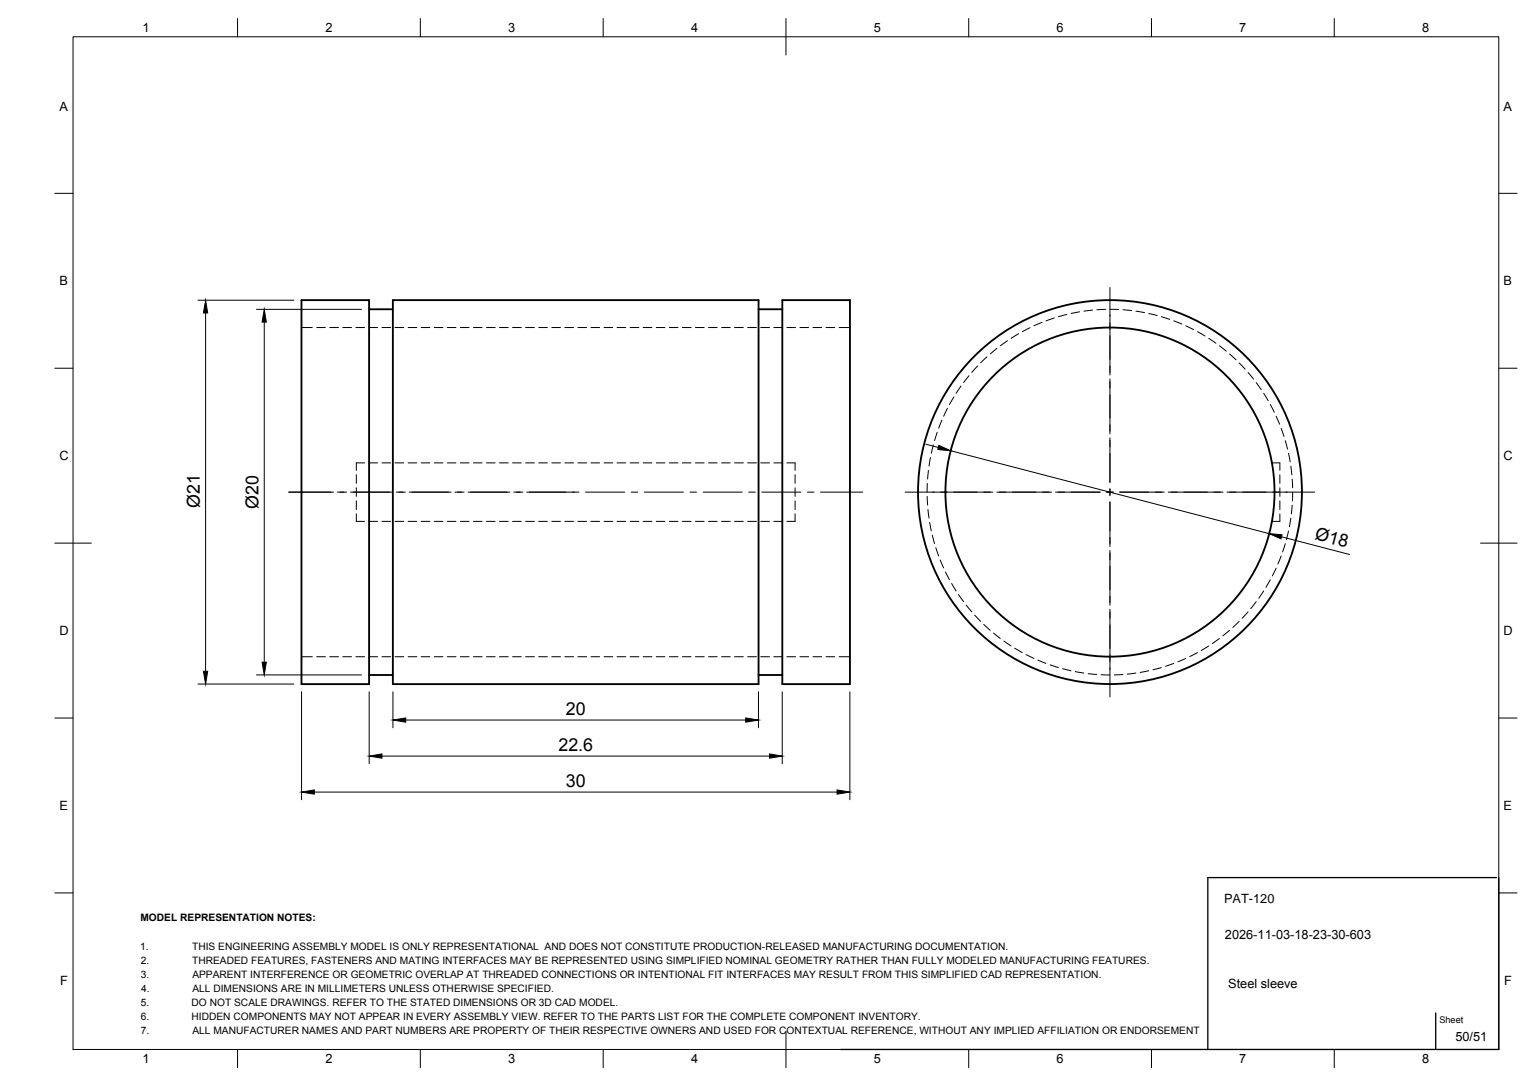
ISO-10303-21;
HEADER;
/* Generated by software containing ST-Developer
 * from STEP Tools, Inc. (www.steptools.com) 
 */

FILE_DESCRIPTION(
/* description */ ('Vibration shaker table dummy'),
/* implementation_level */ '2;1');

FILE_NAME(
/* name */ 'Steel sleeve.step',
/* time_stamp */ '2026-10-27T10:55:14-07:00',
/* author */ (''),
/* organization */ (''),
/* preprocessor_version */ 'ST-DEVELOPER v20.2',
/* originating_system */ 'Autodesk Translation Framework v15.17.0.0',
/* authorisation */ '');

FILE_SCHEMA (('AUTOMOTIVE_DESIGN { 1 0 10303 214 3 1 1 }'));
ENDSEC;

DATA;
#10=MECHANICAL_DESIGN_GEOMETRIC_PRESENTATION_REPRESENTATION('',(#729),#22394);
#637=SHAPE_REPRESENTATION_RELATIONSHIP('SRR','None',#22685,#683);
#683=ADVANCED_BREP_SHAPE_REPRESENTATION('',(#773),#22391);
#729=STYLED_ITEM('',(#22975),#773);
#773=MANIFOLD_SOLID_BREP('Body1',#9249);
#1048=FACE_BOUND('',#2574,.T.);
#1049=FACE_BOUND('',#2577,.T.);
#1050=FACE_BOUND('',#2580,.T.);
#1051=FACE_BOUND('',#2583,.T.);
#1052=FACE_BOUND('',#2586,.T.);
#1053=FACE_BOUND('',#2589,.T.);
#1054=FACE_BOUND('',#2591,.T.);
#1313=PLANE('',#10737);
#1314=PLANE('',#10739);
#1315=PLANE('',#10740);
#1316=PLANE('',#10742);
#1317=PLANE('',#10743);
#1318=PLANE('',#10744);
#1319=PLANE('',#10749);
#1320=PLANE('',#10753);
#1321=PLANE('',#10757);
#1322=PLANE('',#10761);
#1323=PLANE('',#10765);
#1797=FACE_OUTER_BOUND('',#2568,.T.);
#1798=FACE_OUTER_BOUND('',#2569,.T.);
#1799=FACE_OUTER_BOUND('',#2570,.T.);
#1800=FACE_OUTER_BOUND('',#2571,.T.);
#1801=FACE_OUTER_BOUND('',#2572,.T.);
#1802=FACE_OUTER_BOUND('',#2573,.T.);
#1803=FACE_OUTER_BOUND('',#2575,.T.);
#1804=FACE_OUTER_BOUND('',#2576,.T.);
#1805=FACE_OUTER_BOUND('',#2578,.T.);
#1806=FACE_OUTER_BOUND('',#2579,.T.);
#1807=FACE_OUTER_BOUND('',#2581,.T.);
#1808=FACE_OUTER_BOUND('',#2582,.T.);
#1809=FACE_OUTER_BOUND('',#2584,.T.);
#1810=FACE_OUTER_BOUND('',#2585,.T.);
#1811=FACE_OUTER_BOUND('',#2587,.T.);
#1812=FACE_OUTER_BOUND('',#2588,.T.);
#1813=FACE_OUTER_BOUND('',#2590,.T.);
#2568=EDGE_LOOP('',(#8346,#8347,#8348,#8349));
#2569=EDGE_LOOP('',(#8350,#8351,#8352,#8353));
#2570=EDGE_LOOP('',(#8354,#8355,#8356,#8357));
#2571=EDGE_LOOP('',(#8358,#8359,#8360,#8361));
#2572=EDGE_LOOP('',(#8362,#8363,#8364,#8365));
#2573=EDGE_LOOP('',(#8366));
#2574=EDGE_LOOP('',(#8367));
#2575=EDGE_LOOP('',(#8368,#8369,#8370,#8371));
#2576=EDGE_LOOP('',(#8372));
#2577=EDGE_LOOP('',(#8373));
#2578=EDGE_LOOP('',(#8374,#8375,#8376,#8377));
#2579=EDGE_LOOP('',(#8378));
#2580=EDGE_LOOP('',(#8379));
#2581=EDGE_LOOP('',(#8380,#8381,#8382,#8383));
#2582=EDGE_LOOP('',(#8384));
#2583=EDGE_LOOP('',(#8385));
#2584=EDGE_LOOP('',(#8386,#8387,#8388,#8389));
#2585=EDGE_LOOP('',(#8390));
#2586=EDGE_LOOP('',(#8391));
#2587=EDGE_LOOP('',(#8392,#8393,#8394,#8395));
#2588=EDGE_LOOP('',(#8396));
#2589=EDGE_LOOP('',(#8397));
#2590=EDGE_LOOP('',(#8398,#8399,#8400,#8401));
#2591=EDGE_LOOP('',(#8402,#8403,#8404,#8405));
#3191=LINE('',#21983,#3810);
#3192=LINE('',#21985,#3811);
#3193=LINE('',#21986,#3812);
#3194=LINE('',#21989,#3813);
#3195=LINE('',#21991,#3814);
#3196=LINE('',#21992,#3815);
#3197=LINE('',#21997,#3816);
#3198=LINE('',#21998,#3817);
#3199=LINE('',#22000,#3818);
#3200=LINE('',#22001,#3819);
#3201=LINE('',#22011,#3820);
#3202=LINE('',#22018,#3821);
#3203=LINE('',#22025,#3822);
#3204=LINE('',#22032,#3823);
#3205=LINE('',#22039,#3824);
#3206=LINE('',#22044,#3825);
#3810=VECTOR('',#13477,1.);
#3811=VECTOR('',#13478,1.);
#3812=VECTOR('',#13479,1.);
#3813=VECTOR('',#13482,1.);
#3814=VECTOR('',#13483,1.);
#3815=VECTOR('',#13484,1.);
#3816=VECTOR('',#13489,1.);
#3817=VECTOR('',#13490,1.);
#3818=VECTOR('',#13493,1.);
#3819=VECTOR('',#13494,1.);
#3820=VECTOR('',#13507,1.05);
#3821=VECTOR('',#13516,1.);
#3822=VECTOR('',#13525,1.05);
#3823=VECTOR('',#13534,1.);
#3824=VECTOR('',#13543,1.05);
#3825=VECTOR('',#13550,0.9);
#4337=CIRCLE('',#10738,0.9);
#4338=CIRCLE('',#10741,0.9);
#4339=CIRCLE('',#10745,1.05);
#4340=CIRCLE('',#10746,0.9);
#4341=CIRCLE('',#10748,1.05);
#4342=CIRCLE('',#10750,1.);
#4343=CIRCLE('',#10752,1.);
#4344=CIRCLE('',#10754,1.05);
#4345=CIRCLE('',#10756,1.05);
#4346=CIRCLE('',#10758,1.);
#4347=CIRCLE('',#10760,1.);
#4348=CIRCLE('',#10762,1.05);
#4349=CIRCLE('',#10764,1.05);
#4350=CIRCLE('',#10766,0.9);
#5064=VERTEX_POINT('',#21979);
#5065=VERTEX_POINT('',#21980);
#5066=VERTEX_POINT('',#21982);
#5067=VERTEX_POINT('',#21984);
#5068=VERTEX_POINT('',#21988);
#5069=VERTEX_POINT('',#21990);
#5070=VERTEX_POINT('',#21994);
#5071=VERTEX_POINT('',#21996);
#5072=VERTEX_POINT('',#22004);
#5073=VERTEX_POINT('',#22006);
#5074=VERTEX_POINT('',#22009);
#5075=VERTEX_POINT('',#22013);
#5076=VERTEX_POINT('',#22016);
#5077=VERTEX_POINT('',#22020);
#5078=VERTEX_POINT('',#22023);
#5079=VERTEX_POINT('',#22027);
#5080=VERTEX_POINT('',#22030);
#5081=VERTEX_POINT('',#22034);
#5082=VERTEX_POINT('',#22037);
#5083=VERTEX_POINT('',#22041);
#6166=EDGE_CURVE('',#5064,#5065,#4337,.T.);
#6167=EDGE_CURVE('',#5066,#5064,#3191,.T.);
#6168=EDGE_CURVE('',#5067,#5066,#3192,.T.);
#6169=EDGE_CURVE('',#5065,#5067,#3193,.T.);
#6170=EDGE_CURVE('',#5065,#5068,#3194,.T.);
#6171=EDGE_CURVE('',#5069,#5067,#3195,.T.);
#6172=EDGE_CURVE('',#5069,#5068,#3196,.T.);
#6173=EDGE_CURVE('',#5068,#5070,#4338,.T.);
#6174=EDGE_CURVE('',#5071,#5069,#3197,.T.);
#6175=EDGE_CURVE('',#5070,#5071,#3198,.T.);
#6176=EDGE_CURVE('',#5070,#5064,#3199,.T.);
#6177=EDGE_CURVE('',#5071,#5066,#3200,.T.);
#6178=EDGE_CURVE('',#5072,#5072,#4339,.T.);
#6179=EDGE_CURVE('',#5073,#5073,#4340,.T.);
#6180=EDGE_CURVE('',#5074,#5074,#4341,.T.);
#6181=EDGE_CURVE('',#5074,#5072,#3201,.T.);
#6182=EDGE_CURVE('',#5075,#5075,#4342,.T.);
#6183=EDGE_CURVE('',#5076,#5076,#4343,.T.);
#6184=EDGE_CURVE('',#5076,#5075,#3202,.T.);
#6185=EDGE_CURVE('',#5077,#5077,#4344,.T.);
#6186=EDGE_CURVE('',#5078,#5078,#4345,.T.);
#6187=EDGE_CURVE('',#5078,#5077,#3203,.T.);
#6188=EDGE_CURVE('',#5079,#5079,#4346,.T.);
#6189=EDGE_CURVE('',#5080,#5080,#4347,.T.);
#6190=EDGE_CURVE('',#5080,#5079,#3204,.T.);
#6191=EDGE_CURVE('',#5081,#5081,#4348,.T.);
#6192=EDGE_CURVE('',#5082,#5082,#4349,.T.);
#6193=EDGE_CURVE('',#5082,#5081,#3205,.T.);
#6194=EDGE_CURVE('',#5083,#5083,#4350,.T.);
#6195=EDGE_CURVE('',#5083,#5073,#3206,.T.);
#8346=ORIENTED_EDGE('',*,*,#6166,.F.);
#8347=ORIENTED_EDGE('',*,*,#6167,.F.);
#8348=ORIENTED_EDGE('',*,*,#6168,.F.);
#8349=ORIENTED_EDGE('',*,*,#6169,.F.);
#8350=ORIENTED_EDGE('',*,*,#6170,.F.);
#8351=ORIENTED_EDGE('',*,*,#6169,.T.);
#8352=ORIENTED_EDGE('',*,*,#6171,.F.);
#8353=ORIENTED_EDGE('',*,*,#6172,.T.);
#8354=ORIENTED_EDGE('',*,*,#6173,.F.);
#8355=ORIENTED_EDGE('',*,*,#6172,.F.);
#8356=ORIENTED_EDGE('',*,*,#6174,.F.);
#8357=ORIENTED_EDGE('',*,*,#6175,.F.);
#8358=ORIENTED_EDGE('',*,*,#6176,.F.);
#8359=ORIENTED_EDGE('',*,*,#6175,.T.);
#8360=ORIENTED_EDGE('',*,*,#6177,.T.);
#8361=ORIENTED_EDGE('',*,*,#6167,.T.);
#8362=ORIENTED_EDGE('',*,*,#6177,.F.);
#8363=ORIENTED_EDGE('',*,*,#6174,.T.);
#8364=ORIENTED_EDGE('',*,*,#6171,.T.);
#8365=ORIENTED_EDGE('',*,*,#6168,.T.);
#8366=ORIENTED_EDGE('',*,*,#6178,.F.);
#8367=ORIENTED_EDGE('',*,*,#6179,.T.);
#8368=ORIENTED_EDGE('',*,*,#6180,.F.);
#8369=ORIENTED_EDGE('',*,*,#6181,.T.);
#8370=ORIENTED_EDGE('',*,*,#6178,.T.);
#8371=ORIENTED_EDGE('',*,*,#6181,.F.);
#8372=ORIENTED_EDGE('',*,*,#6180,.T.);
#8373=ORIENTED_EDGE('',*,*,#6182,.F.);
#8374=ORIENTED_EDGE('',*,*,#6183,.F.);
#8375=ORIENTED_EDGE('',*,*,#6184,.T.);
#8376=ORIENTED_EDGE('',*,*,#6182,.T.);
#8377=ORIENTED_EDGE('',*,*,#6184,.F.);
#8378=ORIENTED_EDGE('',*,*,#6185,.F.);
#8379=ORIENTED_EDGE('',*,*,#6183,.T.);
#8380=ORIENTED_EDGE('',*,*,#6186,.F.);
#8381=ORIENTED_EDGE('',*,*,#6187,.T.);
#8382=ORIENTED_EDGE('',*,*,#6185,.T.);
#8383=ORIENTED_EDGE('',*,*,#6187,.F.);
#8384=ORIENTED_EDGE('',*,*,#6186,.T.);
#8385=ORIENTED_EDGE('',*,*,#6188,.F.);
#8386=ORIENTED_EDGE('',*,*,#6189,.F.);
#8387=ORIENTED_EDGE('',*,*,#6190,.T.);
#8388=ORIENTED_EDGE('',*,*,#6188,.T.);
#8389=ORIENTED_EDGE('',*,*,#6190,.F.);
#8390=ORIENTED_EDGE('',*,*,#6191,.F.);
#8391=ORIENTED_EDGE('',*,*,#6189,.T.);
#8392=ORIENTED_EDGE('',*,*,#6192,.F.);
#8393=ORIENTED_EDGE('',*,*,#6193,.T.);
#8394=ORIENTED_EDGE('',*,*,#6191,.T.);
#8395=ORIENTED_EDGE('',*,*,#6193,.F.);
#8396=ORIENTED_EDGE('',*,*,#6192,.T.);
#8397=ORIENTED_EDGE('',*,*,#6194,.F.);
#8398=ORIENTED_EDGE('',*,*,#6194,.T.);
#8399=ORIENTED_EDGE('',*,*,#6195,.T.);
#8400=ORIENTED_EDGE('',*,*,#6179,.F.);
#8401=ORIENTED_EDGE('',*,*,#6195,.F.);
#8402=ORIENTED_EDGE('',*,*,#6173,.T.);
#8403=ORIENTED_EDGE('',*,*,#6176,.T.);
#8404=ORIENTED_EDGE('',*,*,#6166,.T.);
#8405=ORIENTED_EDGE('',*,*,#6170,.T.);
#8696=CYLINDRICAL_SURFACE('',#10747,1.05);
#8697=CYLINDRICAL_SURFACE('',#10751,1.);
#8698=CYLINDRICAL_SURFACE('',#10755,1.05);
#8699=CYLINDRICAL_SURFACE('',#10759,1.);
#8700=CYLINDRICAL_SURFACE('',#10763,1.05);
#8701=CYLINDRICAL_SURFACE('',#10767,0.9);
#9162=ADVANCED_FACE('',(#1797),#1313,.F.);
#9163=ADVANCED_FACE('',(#1798),#1314,.F.);
#9164=ADVANCED_FACE('',(#1799),#1315,.F.);
#9165=ADVANCED_FACE('',(#1800),#1316,.F.);
#9166=ADVANCED_FACE('',(#1801),#1317,.F.);
#9167=ADVANCED_FACE('',(#1802,#1048),#1318,.T.);
#9168=ADVANCED_FACE('',(#1803),#8696,.T.);
#9169=ADVANCED_FACE('',(#1804,#1049),#1319,.T.);
#9170=ADVANCED_FACE('',(#1805),#8697,.T.);
#9171=ADVANCED_FACE('',(#1806,#1050),#1320,.T.);
#9172=ADVANCED_FACE('',(#1807),#8698,.T.);
#9173=ADVANCED_FACE('',(#1808,#1051),#1321,.T.);
#9174=ADVANCED_FACE('',(#1809),#8699,.T.);
#9175=ADVANCED_FACE('',(#1810,#1052),#1322,.T.);
#9176=ADVANCED_FACE('',(#1811),#8700,.T.);
#9177=ADVANCED_FACE('',(#1812,#1053),#1323,.T.);
#9178=ADVANCED_FACE('',(#1813,#1054),#8701,.F.);
#9249=CLOSED_SHELL('',(#9162,#9163,#9164,#9165,#9166,#9167,#9168,#9169,
#9170,#9171,#9172,#9173,#9174,#9175,#9176,#9177,#9178));
#10736=AXIS2_PLACEMENT_3D('',#21977,#13471,#13472);
#10737=AXIS2_PLACEMENT_3D('',#21978,#13473,#13474);
#10738=AXIS2_PLACEMENT_3D('',#21981,#13475,#13476);
#10739=AXIS2_PLACEMENT_3D('',#21987,#13480,#13481);
#10740=AXIS2_PLACEMENT_3D('',#21993,#13485,#13486);
#10741=AXIS2_PLACEMENT_3D('',#21995,#13487,#13488);
#10742=AXIS2_PLACEMENT_3D('',#21999,#13491,#13492);
#10743=AXIS2_PLACEMENT_3D('',#22002,#13495,#13496);
#10744=AXIS2_PLACEMENT_3D('',#22003,#13497,#13498);
#10745=AXIS2_PLACEMENT_3D('',#22005,#13499,#13500);
#10746=AXIS2_PLACEMENT_3D('',#22007,#13501,#13502);
#10747=AXIS2_PLACEMENT_3D('',#22008,#13503,#13504);
#10748=AXIS2_PLACEMENT_3D('',#22010,#13505,#13506);
#10749=AXIS2_PLACEMENT_3D('',#22012,#13508,#13509);
#10750=AXIS2_PLACEMENT_3D('',#22014,#13510,#13511);
#10751=AXIS2_PLACEMENT_3D('',#22015,#13512,#13513);
#10752=AXIS2_PLACEMENT_3D('',#22017,#13514,#13515);
#10753=AXIS2_PLACEMENT_3D('',#22019,#13517,#13518);
#10754=AXIS2_PLACEMENT_3D('',#22021,#13519,#13520);
#10755=AXIS2_PLACEMENT_3D('',#22022,#13521,#13522);
#10756=AXIS2_PLACEMENT_3D('',#22024,#13523,#13524);
#10757=AXIS2_PLACEMENT_3D('',#22026,#13526,#13527);
#10758=AXIS2_PLACEMENT_3D('',#22028,#13528,#13529);
#10759=AXIS2_PLACEMENT_3D('',#22029,#13530,#13531);
#10760=AXIS2_PLACEMENT_3D('',#22031,#13532,#13533);
#10761=AXIS2_PLACEMENT_3D('',#22033,#13535,#13536);
#10762=AXIS2_PLACEMENT_3D('',#22035,#13537,#13538);
#10763=AXIS2_PLACEMENT_3D('',#22036,#13539,#13540);
#10764=AXIS2_PLACEMENT_3D('',#22038,#13541,#13542);
#10765=AXIS2_PLACEMENT_3D('',#22040,#13544,#13545);
#10766=AXIS2_PLACEMENT_3D('',#22042,#13546,#13547);
#10767=AXIS2_PLACEMENT_3D('',#22043,#13548,#13549);
#13471=DIRECTION('axis',(0.,0.,1.));
#13472=DIRECTION('refdir',(1.,0.,0.));
#13473=DIRECTION('center_axis',(0.,1.,0.));
#13474=DIRECTION('ref_axis',(0.,0.,1.));
#13475=DIRECTION('center_axis',(0.,-1.,0.));
#13476=DIRECTION('ref_axis',(1.,0.,0.));
#13477=DIRECTION('',(-1.,0.,0.));
#13478=DIRECTION('',(0.,0.,-1.));
#13479=DIRECTION('',(1.,0.,0.));
#13480=DIRECTION('center_axis',(0.,0.,1.));
#13481=DIRECTION('ref_axis',(1.,0.,0.));
#13482=DIRECTION('',(0.,-1.,0.));
#13483=DIRECTION('',(0.,1.,0.));
#13484=DIRECTION('',(-1.,0.,0.));
#13485=DIRECTION('center_axis',(0.,-1.,0.));
#13486=DIRECTION('ref_axis',(0.,0.,-1.));
#13487=DIRECTION('center_axis',(0.,1.,0.));
#13488=DIRECTION('ref_axis',(1.,0.,0.));
#13489=DIRECTION('',(0.,0.,1.));
#13490=DIRECTION('',(1.,0.,0.));
#13491=DIRECTION('center_axis',(0.,0.,-1.));
#13492=DIRECTION('ref_axis',(-1.,0.,0.));
#13493=DIRECTION('',(0.,1.,0.));
#13494=DIRECTION('',(0.,1.,0.));
#13495=DIRECTION('center_axis',(1.,0.,0.));
#13496=DIRECTION('ref_axis',(0.,0.,-1.));
#13497=DIRECTION('center_axis',(0.,1.,0.));
#13498=DIRECTION('ref_axis',(0.,0.,1.));
#13499=DIRECTION('center_axis',(0.,-1.,0.));
#13500=DIRECTION('ref_axis',(1.,0.,0.));
#13501=DIRECTION('center_axis',(0.,-1.,0.));
#13502=DIRECTION('ref_axis',(1.,0.,0.));
#13503=DIRECTION('center_axis',(0.,-1.,0.));
#13504=DIRECTION('ref_axis',(1.,0.,0.));
#13505=DIRECTION('center_axis',(0.,-1.,0.));
#13506=DIRECTION('ref_axis',(1.,0.,0.));
#13507=DIRECTION('',(0.,1.,0.));
#13508=DIRECTION('center_axis',(0.,-1.,0.));
#13509=DIRECTION('ref_axis',(0.,0.,-1.));
#13510=DIRECTION('center_axis',(0.,-1.,0.));
#13511=DIRECTION('ref_axis',(1.,0.,0.));
#13512=DIRECTION('center_axis',(0.,-1.,0.));
#13513=DIRECTION('ref_axis',(1.,0.,0.));
#13514=DIRECTION('center_axis',(0.,-1.,0.));
#13515=DIRECTION('ref_axis',(1.,0.,0.));
#13516=DIRECTION('',(0.,1.,0.));
#13517=DIRECTION('center_axis',(0.,1.,0.));
#13518=DIRECTION('ref_axis',(0.,0.,1.));
#13519=DIRECTION('center_axis',(0.,-1.,0.));
#13520=DIRECTION('ref_axis',(1.,0.,0.));
#13521=DIRECTION('center_axis',(0.,-1.,0.));
#13522=DIRECTION('ref_axis',(1.,0.,0.));
#13523=DIRECTION('center_axis',(0.,-1.,0.));
#13524=DIRECTION('ref_axis',(1.,0.,0.));
#13525=DIRECTION('',(0.,1.,0.));
#13526=DIRECTION('center_axis',(0.,-1.,0.));
#13527=DIRECTION('ref_axis',(0.,0.,-1.));
#13528=DIRECTION('center_axis',(0.,-1.,0.));
#13529=DIRECTION('ref_axis',(1.,0.,0.));
#13530=DIRECTION('center_axis',(0.,-1.,0.));
#13531=DIRECTION('ref_axis',(1.,0.,0.));
#13532=DIRECTION('center_axis',(0.,-1.,0.));
#13533=DIRECTION('ref_axis',(1.,0.,0.));
#13534=DIRECTION('',(0.,1.,0.));
#13535=DIRECTION('center_axis',(0.,1.,0.));
#13536=DIRECTION('ref_axis',(0.,0.,1.));
#13537=DIRECTION('center_axis',(0.,-1.,0.));
#13538=DIRECTION('ref_axis',(1.,0.,0.));
#13539=DIRECTION('center_axis',(0.,-1.,0.));
#13540=DIRECTION('ref_axis',(1.,0.,0.));
#13541=DIRECTION('center_axis',(0.,-1.,0.));
#13542=DIRECTION('ref_axis',(1.,0.,0.));
#13543=DIRECTION('',(0.,1.,0.));
#13544=DIRECTION('center_axis',(0.,-1.,0.));
#13545=DIRECTION('ref_axis',(0.,0.,-1.));
#13546=DIRECTION('center_axis',(0.,-1.,0.));
#13547=DIRECTION('ref_axis',(1.,0.,0.));
#13548=DIRECTION('center_axis',(0.,-1.,0.));
#13549=DIRECTION('ref_axis',(1.,0.,0.));
#13550=DIRECTION('',(0.,1.,0.));
#21977=CARTESIAN_POINT('',(0.,0.,0.));
#21978=CARTESIAN_POINT('Origin',(0.75,1.2,0.));
#21979=CARTESIAN_POINT('',(0.885663593019381,1.2,-0.16));
#21980=CARTESIAN_POINT('',(0.885663593019381,1.2,0.16));
#21981=CARTESIAN_POINT('Origin',(0.,1.2,0.));
#21982=CARTESIAN_POINT('',(0.93,1.2,-0.16));
#21983=CARTESIAN_POINT('',(0.93,1.2,-0.16));
#21984=CARTESIAN_POINT('',(0.93,1.2,0.16));
#21985=CARTESIAN_POINT('',(0.93,1.2,0.16));
#21986=CARTESIAN_POINT('',(0.57,1.2,0.16));
#21987=CARTESIAN_POINT('Origin',(0.57,0.,0.16));
#21988=CARTESIAN_POINT('',(0.885663593019381,-1.2,0.16));
#21989=CARTESIAN_POINT('',(0.885663593019381,0.,0.16));
#21990=CARTESIAN_POINT('',(0.93,-1.2,0.16));
#21991=CARTESIAN_POINT('',(0.93,0.,0.16));
#21992=CARTESIAN_POINT('',(0.57,-1.2,0.16));
#21993=CARTESIAN_POINT('Origin',(0.75,-1.2,0.));
#21994=CARTESIAN_POINT('',(0.885663593019381,-1.2,-0.16));
#21995=CARTESIAN_POINT('Origin',(0.,-1.2,0.));
#21996=CARTESIAN_POINT('',(0.93,-1.2,-0.16));
#21997=CARTESIAN_POINT('',(0.93,-1.2,0.16));
#21998=CARTESIAN_POINT('',(0.93,-1.2,-0.16));
#21999=CARTESIAN_POINT('Origin',(0.93,0.,-0.16));
#22000=CARTESIAN_POINT('',(0.885663593019381,0.,-0.16));
#22001=CARTESIAN_POINT('',(0.93,0.,-0.16));
#22002=CARTESIAN_POINT('Origin',(0.93,0.,0.16));
#22003=CARTESIAN_POINT('Origin',(1.05,1.5,0.));
#22004=CARTESIAN_POINT('',(-1.05,1.5,-1.28587913910472E-16));
#22005=CARTESIAN_POINT('Origin',(0.,1.5,0.));
#22006=CARTESIAN_POINT('',(-0.9,1.5,-1.10218211923262E-16));
#22007=CARTESIAN_POINT('Origin',(0.,1.5,0.));
#22008=CARTESIAN_POINT('Origin',(0.,1.315,0.));
#22009=CARTESIAN_POINT('',(-1.05,1.13,-1.28587913910472E-16));
#22010=CARTESIAN_POINT('Origin',(0.,1.13,0.));
#22011=CARTESIAN_POINT('',(-1.05,1.315,-1.28587913910472E-16));
#22012=CARTESIAN_POINT('Origin',(1.,1.13,0.));
#22013=CARTESIAN_POINT('',(-1.,1.13,-1.22464679914735E-16));
#22014=CARTESIAN_POINT('Origin',(0.,1.13,0.));
#22015=CARTESIAN_POINT('Origin',(0.,1.065,0.));
#22016=CARTESIAN_POINT('',(-1.,1.,-1.22464679914735E-16));
#22017=CARTESIAN_POINT('Origin',(0.,1.,0.));
#22018=CARTESIAN_POINT('',(-1.,1.065,-1.22464679914735E-16));
#22019=CARTESIAN_POINT('Origin',(1.05,1.,0.));
#22020=CARTESIAN_POINT('',(-1.05,1.,-1.28587913910472E-16));
#22021=CARTESIAN_POINT('Origin',(0.,1.,0.));
#22022=CARTESIAN_POINT('Origin',(0.,0.,0.));
#22023=CARTESIAN_POINT('',(-1.05,-1.,-1.28587913910472E-16));
#22024=CARTESIAN_POINT('Origin',(0.,-1.,0.));
#22025=CARTESIAN_POINT('',(-1.05,0.,-1.28587913910472E-16));
#22026=CARTESIAN_POINT('Origin',(1.,-1.,0.));
#22027=CARTESIAN_POINT('',(-1.,-1.,-1.22464679914735E-16));
#22028=CARTESIAN_POINT('Origin',(0.,-1.,0.));
#22029=CARTESIAN_POINT('Origin',(0.,-1.065,0.));
#22030=CARTESIAN_POINT('',(-1.,-1.13,-1.22464679914735E-16));
#22031=CARTESIAN_POINT('Origin',(0.,-1.13,0.));
#22032=CARTESIAN_POINT('',(-1.,-1.065,-1.22464679914735E-16));
#22033=CARTESIAN_POINT('Origin',(1.05,-1.13,0.));
#22034=CARTESIAN_POINT('',(-1.05,-1.13,-1.28587913910472E-16));
#22035=CARTESIAN_POINT('Origin',(0.,-1.13,0.));
#22036=CARTESIAN_POINT('Origin',(0.,-1.315,0.));
#22037=CARTESIAN_POINT('',(-1.05,-1.5,-1.28587913910472E-16));
#22038=CARTESIAN_POINT('Origin',(0.,-1.5,0.));
#22039=CARTESIAN_POINT('',(-1.05,-1.315,-1.28587913910472E-16));
#22040=CARTESIAN_POINT('Origin',(0.9,-1.5,0.));
#22041=CARTESIAN_POINT('',(-0.9,-1.5,-1.10218211923262E-16));
#22042=CARTESIAN_POINT('Origin',(0.,-1.5,0.));
#22043=CARTESIAN_POINT('Origin',(0.,0.,0.));
#22044=CARTESIAN_POINT('',(-0.9,0.,-1.10218211923262E-16));
#22340=UNCERTAINTY_MEASURE_WITH_UNIT(LENGTH_MEASURE(0.001),#22395,
'DISTANCE_ACCURACY_VALUE',
'Maximum model space distance between geometric entities at asserted c
onnectivities');
#22343=UNCERTAINTY_MEASURE_WITH_UNIT(LENGTH_MEASURE(0.001),#22395,
'DISTANCE_ACCURACY_VALUE',
'Maximum model space distance between geometric entities at asserted c
onnectivities');
#22391=(
GEOMETRIC_REPRESENTATION_CONTEXT(3)
GLOBAL_UNCERTAINTY_ASSIGNED_CONTEXT((#22340))
GLOBAL_UNIT_ASSIGNED_CONTEXT((#22395,#22397,#22398))
REPRESENTATION_CONTEXT('','3D')
);
#22394=(
GEOMETRIC_REPRESENTATION_CONTEXT(3)
GLOBAL_UNCERTAINTY_ASSIGNED_CONTEXT((#22343))
GLOBAL_UNIT_ASSIGNED_CONTEXT((#22395,#22397,#22398))
REPRESENTATION_CONTEXT('','3D')
);
#22395=(
LENGTH_UNIT()
NAMED_UNIT(*)
SI_UNIT(.CENTI.,.METRE.)
);
#22397=(
NAMED_UNIT(*)
PLANE_ANGLE_UNIT()
SI_UNIT($,.RADIAN.)
);
#22398=(
NAMED_UNIT(*)
SI_UNIT($,.STERADIAN.)
SOLID_ANGLE_UNIT()
);
#22446=SHAPE_DEFINITION_REPRESENTATION(#22496,#22685);
#22496=PRODUCT_DEFINITION_SHAPE('',$,#22736);
#22685=SHAPE_REPRESENTATION('',(#10736),#22391);
#22688=PRODUCT_DEFINITION_CONTEXT('part definition',#22840,'design');
#22736=PRODUCT_DEFINITION('Steel sleeve','Steel sleeve',#22786,#22688);
#22786=PRODUCT_DEFINITION_FORMATION('',$,#22889);
#22840=APPLICATION_CONTEXT(
'Core Data for Automotive Mechanical Design Process');
#22841=PRODUCT_CONTEXT('part definition',#22840,'mechanical');
#22889=PRODUCT('Steel sleeve','Steel sleeve','Steel sleeve',(#22841));
#22969=COLOUR_RGB('Off White',0.89,0.88,0.83);
#22970=FILL_AREA_STYLE_COLOUR('',#22969);
#22971=FILL_AREA_STYLE('',(#22970));
#22972=SURFACE_STYLE_FILL_AREA(#22971);
#22973=SURFACE_SIDE_STYLE('',(#22972));
#22974=SURFACE_STYLE_USAGE(.BOTH.,#22973);
#22975=PRESENTATION_STYLE_ASSIGNMENT((#22974));
ENDSEC;
END-ISO-10303-21;
